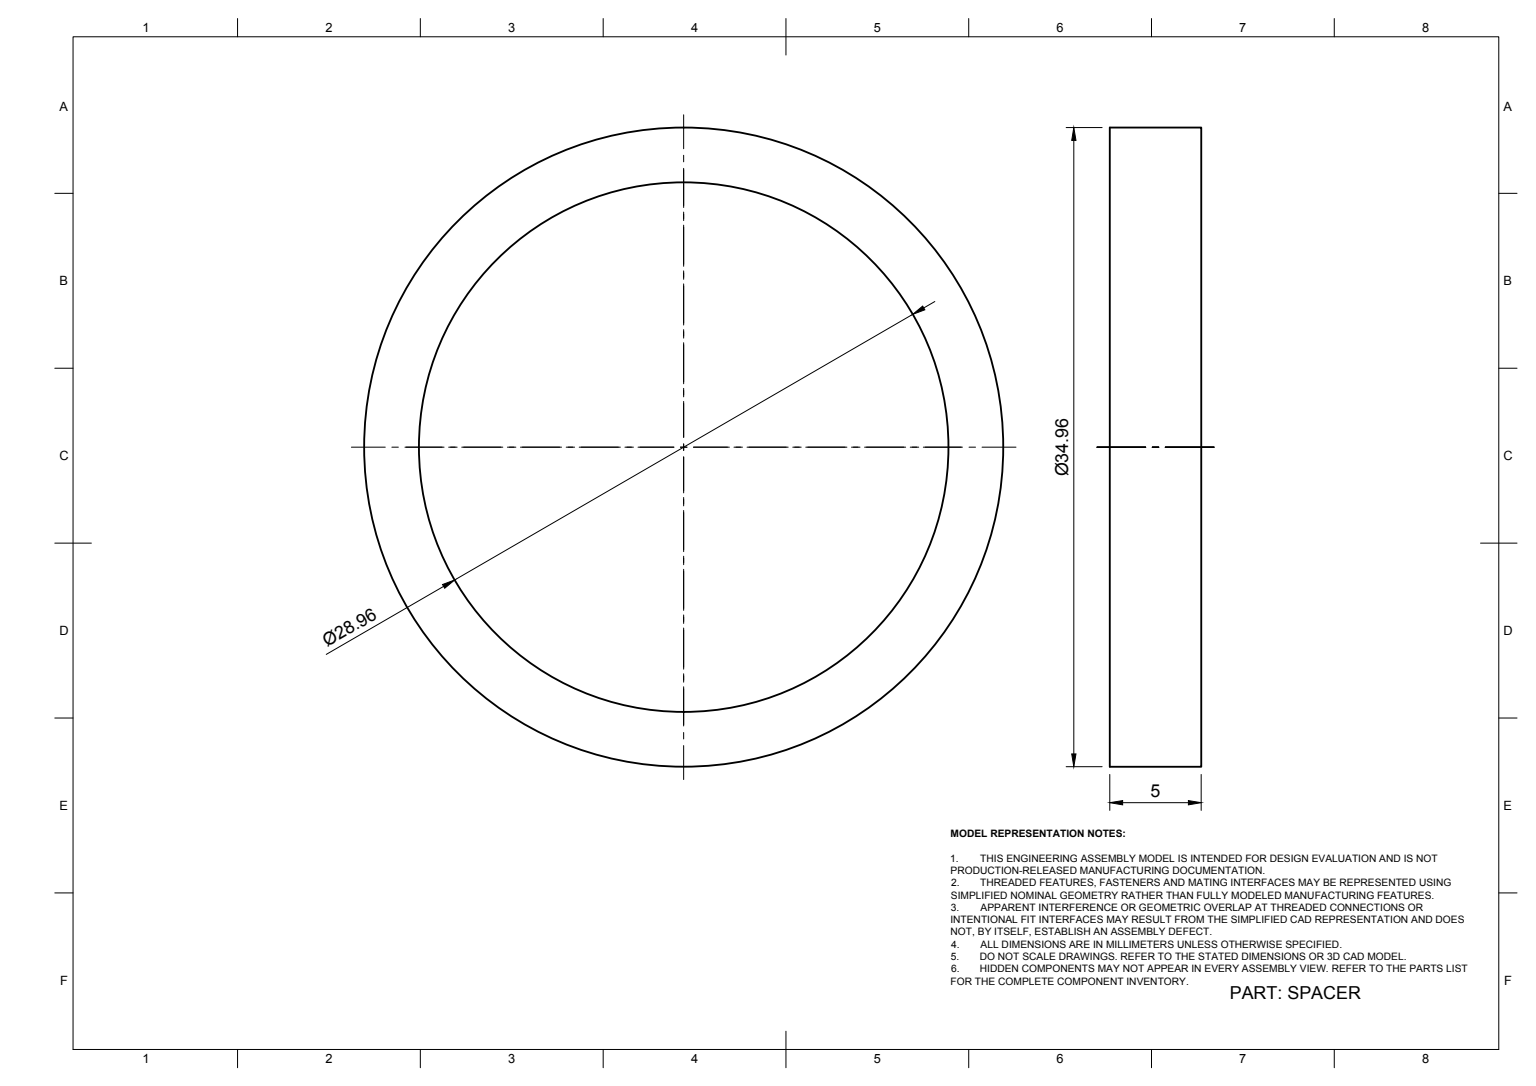
ISO-10303-21;
HEADER;
/* Generated by software containing ST-Developer
 * from STEP Tools, Inc. (www.steptools.com) 
 */

FILE_DESCRIPTION(
/* description */ (''),
/* implementation_level */ '2;1');

FILE_NAME(
/* name */ 'Spacer.step',
/* time_stamp */ '2026-09-20T22:38:01+06:00',
/* author */ (''),
/* organization */ (''),
/* preprocessor_version */ 'ST-DEVELOPER v20.2',
/* originating_system */ 'Autodesk Translation Framework v15.15.0.0',
/* authorisation */ '');

FILE_SCHEMA (('AUTOMOTIVE_DESIGN { 1 0 10303 214 3 1 1 }'));
ENDSEC;

DATA;
#10=MECHANICAL_DESIGN_GEOMETRIC_PRESENTATION_REPRESENTATION('',(#87),#4079);
#71=SHAPE_REPRESENTATION_RELATIONSHIP('SRR','None',#4114,#79);
#79=ADVANCED_BREP_SHAPE_REPRESENTATION('',(#95),#4074);
#87=STYLED_ITEM('',(#4159),#95);
#95=MANIFOLD_SOLID_BREP('Spacer',#1446);
#104=FACE_BOUND('',#348,.T.);
#105=FACE_BOUND('',#350,.T.);
#157=CIRCLE('',#1651,14.4819556358054);
#158=CIRCLE('',#1652,14.4819556358054);
#159=CIRCLE('',#1654,17.4819556358054);
#160=CIRCLE('',#1655,17.4819556358054);
#191=CYLINDRICAL_SURFACE('',#1650,14.4819556358054);
#192=CYLINDRICAL_SURFACE('',#1653,17.4819556358054);
#257=FACE_OUTER_BOUND('',#345,.T.);
#258=FACE_OUTER_BOUND('',#346,.T.);
#259=FACE_OUTER_BOUND('',#347,.T.);
#260=FACE_OUTER_BOUND('',#349,.T.);
#345=EDGE_LOOP('',(#1225,#1226,#1227,#1228));
#346=EDGE_LOOP('',(#1229,#1230,#1231,#1232));
#347=EDGE_LOOP('',(#1233));
#348=EDGE_LOOP('',(#1234));
#349=EDGE_LOOP('',(#1235));
#350=EDGE_LOOP('',(#1236));
#454=LINE('',#3958,#567);
#455=LINE('',#3964,#568);
#567=VECTOR('',#2005,14.4819556358054);
#568=VECTOR('',#2012,17.4819556358054);
#696=VERTEX_POINT('',#3955);
#697=VERTEX_POINT('',#3957);
#698=VERTEX_POINT('',#3961);
#699=VERTEX_POINT('',#3963);
#877=EDGE_CURVE('',#696,#696,#157,.T.);
#878=EDGE_CURVE('',#696,#697,#454,.T.);
#879=EDGE_CURVE('',#697,#697,#158,.T.);
#880=EDGE_CURVE('',#698,#698,#159,.T.);
#881=EDGE_CURVE('',#698,#699,#455,.T.);
#882=EDGE_CURVE('',#699,#699,#160,.T.);
#1225=ORIENTED_EDGE('',*,*,#877,.F.);
#1226=ORIENTED_EDGE('',*,*,#878,.T.);
#1227=ORIENTED_EDGE('',*,*,#879,.T.);
#1228=ORIENTED_EDGE('',*,*,#878,.F.);
#1229=ORIENTED_EDGE('',*,*,#880,.F.);
#1230=ORIENTED_EDGE('',*,*,#881,.T.);
#1231=ORIENTED_EDGE('',*,*,#882,.T.);
#1232=ORIENTED_EDGE('',*,*,#881,.F.);
#1233=ORIENTED_EDGE('',*,*,#880,.T.);
#1234=ORIENTED_EDGE('',*,*,#877,.T.);
#1235=ORIENTED_EDGE('',*,*,#882,.F.);
#1236=ORIENTED_EDGE('',*,*,#879,.F.);
#1341=PLANE('',#1656);
#1342=PLANE('',#1657);
#1419=ADVANCED_FACE('',(#257),#191,.F.);
#1420=ADVANCED_FACE('',(#258),#192,.T.);
#1421=ADVANCED_FACE('',(#259,#104),#1341,.T.);
#1422=ADVANCED_FACE('',(#260,#105),#1342,.F.);
#1446=CLOSED_SHELL('',(#1419,#1420,#1421,#1422));
#1649=AXIS2_PLACEMENT_3D('',#3953,#1999,#2000);
#1650=AXIS2_PLACEMENT_3D('',#3954,#2001,#2002);
#1651=AXIS2_PLACEMENT_3D('',#3956,#2003,#2004);
#1652=AXIS2_PLACEMENT_3D('',#3959,#2006,#2007);
#1653=AXIS2_PLACEMENT_3D('',#3960,#2008,#2009);
#1654=AXIS2_PLACEMENT_3D('',#3962,#2010,#2011);
#1655=AXIS2_PLACEMENT_3D('',#3965,#2013,#2014);
#1656=AXIS2_PLACEMENT_3D('',#3966,#2015,#2016);
#1657=AXIS2_PLACEMENT_3D('',#3967,#2017,#2018);
#1999=DIRECTION('axis',(0.,0.,1.));
#2000=DIRECTION('refdir',(1.,0.,0.));
#2001=DIRECTION('center_axis',(0.,-1.,0.));
#2002=DIRECTION('ref_axis',(1.,0.,0.));
#2003=DIRECTION('center_axis',(0.,1.,0.));
#2004=DIRECTION('ref_axis',(1.,0.,0.));
#2005=DIRECTION('',(0.,1.,0.));
#2006=DIRECTION('center_axis',(0.,1.,0.));
#2007=DIRECTION('ref_axis',(1.,0.,0.));
#2008=DIRECTION('center_axis',(0.,-1.,0.));
#2009=DIRECTION('ref_axis',(1.,0.,0.));
#2010=DIRECTION('center_axis',(0.,-1.,0.));
#2011=DIRECTION('ref_axis',(1.,0.,0.));
#2012=DIRECTION('',(0.,1.,0.));
#2013=DIRECTION('center_axis',(0.,-1.,0.));
#2014=DIRECTION('ref_axis',(1.,0.,0.));
#2015=DIRECTION('center_axis',(0.,-1.,0.));
#2016=DIRECTION('ref_axis',(1.,0.,0.));
#2017=DIRECTION('center_axis',(0.,-1.,0.));
#2018=DIRECTION('ref_axis',(1.,0.,0.));
#3953=CARTESIAN_POINT('',(0.,0.,0.));
#3954=CARTESIAN_POINT('Origin',(-0.00360820116592981,5.,47.167824608198));
#3955=CARTESIAN_POINT('',(-14.4855638369713,0.,47.167824608198));
#3956=CARTESIAN_POINT('Origin',(-0.00360820116592981,0.,47.167824608198));
#3957=CARTESIAN_POINT('',(-14.4855638369713,5.,47.167824608198));
#3958=CARTESIAN_POINT('',(-14.4855638369713,5.,47.167824608198));
#3959=CARTESIAN_POINT('Origin',(-0.00360820116592981,5.,47.167824608198));
#3960=CARTESIAN_POINT('Origin',(-0.00360820116592981,5.,47.167824608198));
#3961=CARTESIAN_POINT('',(-17.4855638369713,0.,47.167824608198));
#3962=CARTESIAN_POINT('Origin',(-0.00360820116592981,0.,47.167824608198));
#3963=CARTESIAN_POINT('',(-17.4855638369713,5.,47.167824608198));
#3964=CARTESIAN_POINT('',(-17.4855638369713,5.,47.167824608198));
#3965=CARTESIAN_POINT('Origin',(-0.00360820116592981,5.,47.167824608198));
#3966=CARTESIAN_POINT('Origin',(-0.00360820116592997,0.,47.167824608198));
#3967=CARTESIAN_POINT('Origin',(-0.00360820116592997,5.,47.167824608198));
#4064=UNCERTAINTY_MEASURE_WITH_UNIT(LENGTH_MEASURE(0.01),#4080,
'DISTANCE_ACCURACY_VALUE',
'Maximum model space distance between geometric entities at asserted c
onnectivities');
#4069=UNCERTAINTY_MEASURE_WITH_UNIT(LENGTH_MEASURE(0.01),#4080,
'DISTANCE_ACCURACY_VALUE',
'Maximum model space distance between geometric entities at asserted c
onnectivities');
#4074=(
GEOMETRIC_REPRESENTATION_CONTEXT(3)
GLOBAL_UNCERTAINTY_ASSIGNED_CONTEXT((#4064))
GLOBAL_UNIT_ASSIGNED_CONTEXT((#4080,#4082,#4083))
REPRESENTATION_CONTEXT('','3D')
);
#4079=(
GEOMETRIC_REPRESENTATION_CONTEXT(3)
GLOBAL_UNCERTAINTY_ASSIGNED_CONTEXT((#4069))
GLOBAL_UNIT_ASSIGNED_CONTEXT((#4080,#4082,#4083))
REPRESENTATION_CONTEXT('','3D')
);
#4080=(
LENGTH_UNIT()
NAMED_UNIT(*)
SI_UNIT(.MILLI.,.METRE.)
);
#4082=(
NAMED_UNIT(*)
PLANE_ANGLE_UNIT()
SI_UNIT($,.RADIAN.)
);
#4083=(
NAMED_UNIT(*)
SI_UNIT($,.STERADIAN.)
SOLID_ANGLE_UNIT()
);
#4088=SHAPE_DEFINITION_REPRESENTATION(#4097,#4114);
#4097=PRODUCT_DEFINITION_SHAPE('',$,#4124);
#4114=SHAPE_REPRESENTATION('',(#1649),#4074);
#4119=PRODUCT_DEFINITION_CONTEXT('part definition',#4148,'design');
#4124=PRODUCT_DEFINITION('Spacer','Spacer',#4133,#4119);
#4133=PRODUCT_DEFINITION_FORMATION('',$,#4154);
#4148=APPLICATION_CONTEXT(
'Core Data for Automotive Mechanical Design Process');
#4149=PRODUCT_CONTEXT('part definition',#4148,'mechanical');
#4154=PRODUCT('Spacer','Spacer',$,(#4149));
#4159=PRESENTATION_STYLE_ASSIGNMENT((#4163));
#4163=SURFACE_STYLE_USAGE(.BOTH.,#4167);
#4167=SURFACE_SIDE_STYLE('',(#4171));
#4171=SURFACE_STYLE_FILL_AREA(#4175);
#4175=FILL_AREA_STYLE('Steel - Satin',(#4179));
#4179=FILL_AREA_STYLE_COLOUR('Steel - Satin',#4183);
#4183=COLOUR_RGB('Steel - Satin', 0.40784314, 0.44705882, 0.49803922);
ENDSEC;
END-ISO-10303-21;
